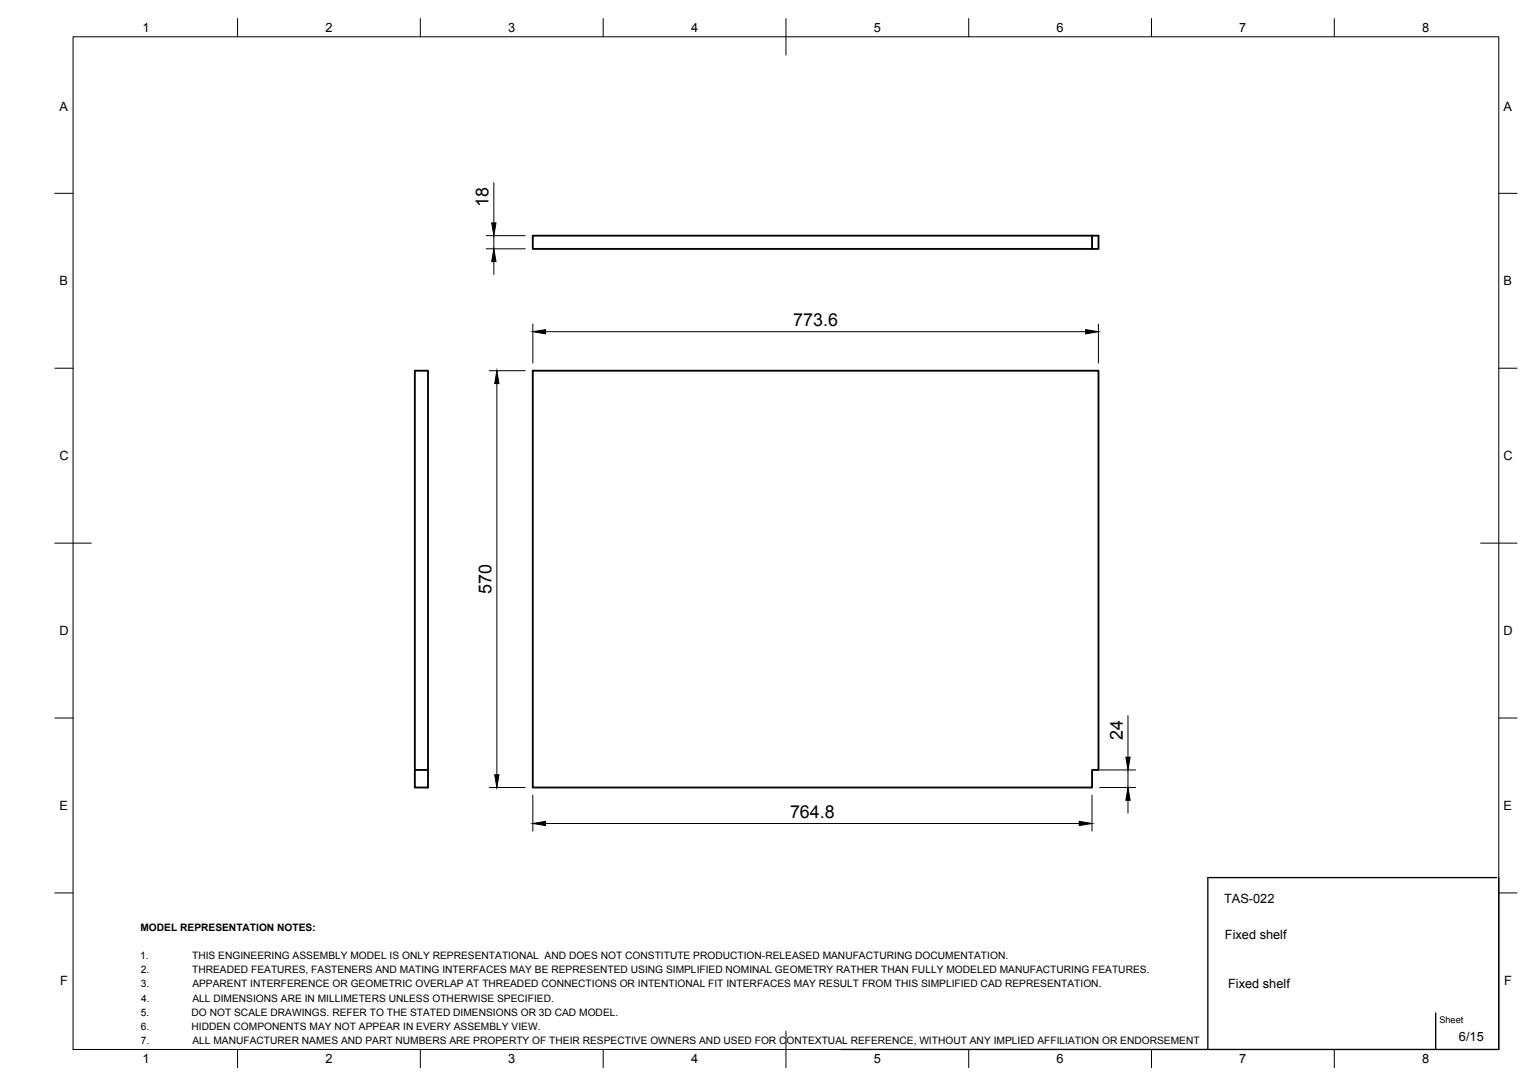
ISO-10303-21;
HEADER;
/* Generated by software containing ST-Developer
 * from STEP Tools, Inc. (www.steptools.com) 
 */

FILE_DESCRIPTION(
/* description */ (''),
/* implementation_level */ '2;1');

FILE_NAME(
/* name */ 'Fixed shelf.step',
/* time_stamp */ '2026-11-15T21:02:08-08:00',
/* author */ (''),
/* organization */ (''),
/* preprocessor_version */ 'ST-DEVELOPER v20.2',
/* originating_system */ 'Autodesk Translation Framework v15.17.0.0',
/* authorisation */ '');

FILE_SCHEMA (('AUTOMOTIVE_DESIGN { 1 0 10303 214 3 1 1 }'));
ENDSEC;

DATA;
#10=MECHANICAL_DESIGN_GEOMETRIC_PRESENTATION_REPRESENTATION('',(#610),#31566);
#580=SHAPE_REPRESENTATION_RELATIONSHIP('SRR','None',#31644,#595);
#595=ADVANCED_BREP_SHAPE_REPRESENTATION('',(#625),#31559);
#610=STYLED_ITEM('',(#31721),#625);
#625=MANIFOLD_SOLID_BREP('Body1',#5723);
#755=FACE_OUTER_BOUND('',#1052,.T.);
#756=FACE_OUTER_BOUND('',#1053,.T.);
#757=FACE_OUTER_BOUND('',#1054,.T.);
#758=FACE_OUTER_BOUND('',#1055,.T.);
#759=FACE_OUTER_BOUND('',#1056,.T.);
#760=FACE_OUTER_BOUND('',#1057,.T.);
#761=FACE_OUTER_BOUND('',#1058,.T.);
#762=FACE_OUTER_BOUND('',#1059,.T.);
#1052=EDGE_LOOP('',(#4245,#4246,#4247,#4248));
#1053=EDGE_LOOP('',(#4249,#4250,#4251,#4252));
#1054=EDGE_LOOP('',(#4253,#4254,#4255,#4256));
#1055=EDGE_LOOP('',(#4257,#4258,#4259,#4260));
#1056=EDGE_LOOP('',(#4261,#4262,#4263,#4264));
#1057=EDGE_LOOP('',(#4265,#4266,#4267,#4268));
#1058=EDGE_LOOP('',(#4269,#4270,#4271,#4272,#4273,#4274));
#1059=EDGE_LOOP('',(#4275,#4276,#4277,#4278,#4279,#4280));
#1463=LINE('',#8212,#1970);
#1464=LINE('',#8214,#1971);
#1465=LINE('',#8216,#1972);
#1466=LINE('',#8217,#1973);
#1467=LINE('',#8220,#1974);
#1468=LINE('',#8222,#1975);
#1469=LINE('',#8223,#1976);
#1470=LINE('',#8226,#1977);
#1471=LINE('',#8228,#1978);
#1472=LINE('',#8229,#1979);
#1473=LINE('',#8232,#1980);
#1474=LINE('',#8234,#1981);
#1475=LINE('',#8235,#1982);
#1476=LINE('',#8238,#1983);
#1477=LINE('',#8240,#1984);
#1478=LINE('',#8241,#1985);
#1479=LINE('',#8243,#1986);
#1480=LINE('',#8244,#1987);
#1970=VECTOR('',#6911,1.);
#1971=VECTOR('',#6912,1.);
#1972=VECTOR('',#6913,1.);
#1973=VECTOR('',#6914,1.);
#1974=VECTOR('',#6917,1.);
#1975=VECTOR('',#6918,1.);
#1976=VECTOR('',#6919,1.);
#1977=VECTOR('',#6922,1.);
#1978=VECTOR('',#6923,1.);
#1979=VECTOR('',#6924,1.);
#1980=VECTOR('',#6927,1.);
#1981=VECTOR('',#6928,1.);
#1982=VECTOR('',#6929,1.);
#1983=VECTOR('',#6932,1.);
#1984=VECTOR('',#6933,1.);
#1985=VECTOR('',#6934,1.);
#1986=VECTOR('',#6937,1.);
#1987=VECTOR('',#6938,1.);
#2426=VERTEX_POINT('',#8210);
#2427=VERTEX_POINT('',#8211);
#2428=VERTEX_POINT('',#8213);
#2429=VERTEX_POINT('',#8215);
#2430=VERTEX_POINT('',#8219);
#2431=VERTEX_POINT('',#8221);
#2432=VERTEX_POINT('',#8225);
#2433=VERTEX_POINT('',#8227);
#2434=VERTEX_POINT('',#8231);
#2435=VERTEX_POINT('',#8233);
#2436=VERTEX_POINT('',#8237);
#2437=VERTEX_POINT('',#8239);
#3118=EDGE_CURVE('',#2426,#2427,#1463,.T.);
#3119=EDGE_CURVE('',#2426,#2428,#1464,.T.);
#3120=EDGE_CURVE('',#2429,#2428,#1465,.T.);
#3121=EDGE_CURVE('',#2427,#2429,#1466,.T.);
#3122=EDGE_CURVE('',#2430,#2426,#1467,.T.);
#3123=EDGE_CURVE('',#2431,#2430,#1468,.T.);
#3124=EDGE_CURVE('',#2428,#2431,#1469,.T.);
#3125=EDGE_CURVE('',#2432,#2429,#1470,.T.);
#3126=EDGE_CURVE('',#2433,#2432,#1471,.T.);
#3127=EDGE_CURVE('',#2433,#2427,#1472,.T.);
#3128=EDGE_CURVE('',#2430,#2434,#1473,.T.);
#3129=EDGE_CURVE('',#2434,#2435,#1474,.T.);
#3130=EDGE_CURVE('',#2431,#2435,#1475,.T.);
#3131=EDGE_CURVE('',#2436,#2433,#1476,.T.);
#3132=EDGE_CURVE('',#2437,#2432,#1477,.T.);
#3133=EDGE_CURVE('',#2436,#2437,#1478,.T.);
#3134=EDGE_CURVE('',#2434,#2436,#1479,.T.);
#3135=EDGE_CURVE('',#2435,#2437,#1480,.T.);
#4245=ORIENTED_EDGE('',*,*,#3118,.F.);
#4246=ORIENTED_EDGE('',*,*,#3119,.T.);
#4247=ORIENTED_EDGE('',*,*,#3120,.F.);
#4248=ORIENTED_EDGE('',*,*,#3121,.F.);
#4249=ORIENTED_EDGE('',*,*,#3122,.F.);
#4250=ORIENTED_EDGE('',*,*,#3123,.F.);
#4251=ORIENTED_EDGE('',*,*,#3124,.F.);
#4252=ORIENTED_EDGE('',*,*,#3119,.F.);
#4253=ORIENTED_EDGE('',*,*,#3121,.T.);
#4254=ORIENTED_EDGE('',*,*,#3125,.F.);
#4255=ORIENTED_EDGE('',*,*,#3126,.F.);
#4256=ORIENTED_EDGE('',*,*,#3127,.T.);
#4257=ORIENTED_EDGE('',*,*,#3123,.T.);
#4258=ORIENTED_EDGE('',*,*,#3128,.T.);
#4259=ORIENTED_EDGE('',*,*,#3129,.T.);
#4260=ORIENTED_EDGE('',*,*,#3130,.F.);
#4261=ORIENTED_EDGE('',*,*,#3131,.T.);
#4262=ORIENTED_EDGE('',*,*,#3126,.T.);
#4263=ORIENTED_EDGE('',*,*,#3132,.F.);
#4264=ORIENTED_EDGE('',*,*,#3133,.F.);
#4265=ORIENTED_EDGE('',*,*,#3134,.T.);
#4266=ORIENTED_EDGE('',*,*,#3133,.T.);
#4267=ORIENTED_EDGE('',*,*,#3135,.F.);
#4268=ORIENTED_EDGE('',*,*,#3129,.F.);
#4269=ORIENTED_EDGE('',*,*,#3124,.T.);
#4270=ORIENTED_EDGE('',*,*,#3130,.T.);
#4271=ORIENTED_EDGE('',*,*,#3135,.T.);
#4272=ORIENTED_EDGE('',*,*,#3132,.T.);
#4273=ORIENTED_EDGE('',*,*,#3125,.T.);
#4274=ORIENTED_EDGE('',*,*,#3120,.T.);
#4275=ORIENTED_EDGE('',*,*,#3118,.T.);
#4276=ORIENTED_EDGE('',*,*,#3127,.F.);
#4277=ORIENTED_EDGE('',*,*,#3131,.F.);
#4278=ORIENTED_EDGE('',*,*,#3134,.F.);
#4279=ORIENTED_EDGE('',*,*,#3128,.F.);
#4280=ORIENTED_EDGE('',*,*,#3122,.T.);
#5360=PLANE('',#6081);
#5361=PLANE('',#6082);
#5362=PLANE('',#6083);
#5363=PLANE('',#6084);
#5364=PLANE('',#6085);
#5365=PLANE('',#6086);
#5366=PLANE('',#6087);
#5367=PLANE('',#6088);
#5569=ADVANCED_FACE('',(#755),#5360,.F.);
#5570=ADVANCED_FACE('',(#756),#5361,.F.);
#5571=ADVANCED_FACE('',(#757),#5362,.T.);
#5572=ADVANCED_FACE('',(#758),#5363,.T.);
#5573=ADVANCED_FACE('',(#759),#5364,.T.);
#5574=ADVANCED_FACE('',(#760),#5365,.T.);
#5575=ADVANCED_FACE('',(#761),#5366,.T.);
#5576=ADVANCED_FACE('',(#762),#5367,.F.);
#5723=CLOSED_SHELL('',(#5569,#5570,#5571,#5572,#5573,#5574,#5575,#5576));
#6080=AXIS2_PLACEMENT_3D('',#8208,#6907,#6908);
#6081=AXIS2_PLACEMENT_3D('',#8209,#6909,#6910);
#6082=AXIS2_PLACEMENT_3D('',#8218,#6915,#6916);
#6083=AXIS2_PLACEMENT_3D('',#8224,#6920,#6921);
#6084=AXIS2_PLACEMENT_3D('',#8230,#6925,#6926);
#6085=AXIS2_PLACEMENT_3D('',#8236,#6930,#6931);
#6086=AXIS2_PLACEMENT_3D('',#8242,#6935,#6936);
#6087=AXIS2_PLACEMENT_3D('',#8245,#6939,#6940);
#6088=AXIS2_PLACEMENT_3D('',#8246,#6941,#6942);
#6907=DIRECTION('axis',(0.,0.,1.));
#6908=DIRECTION('refdir',(1.,0.,0.));
#6909=DIRECTION('center_axis',(0.,1.,0.));
#6910=DIRECTION('ref_axis',(-1.,0.,0.));
#6911=DIRECTION('',(-1.,0.,0.));
#6912=DIRECTION('',(0.,0.,1.));
#6913=DIRECTION('',(1.,0.,0.));
#6914=DIRECTION('',(0.,0.,1.));
#6915=DIRECTION('center_axis',(1.,0.,0.));
#6916=DIRECTION('ref_axis',(0.,1.,0.));
#6917=DIRECTION('',(0.,1.,0.));
#6918=DIRECTION('',(0.,0.,-1.));
#6919=DIRECTION('',(0.,-1.,0.));
#6920=DIRECTION('center_axis',(-1.,0.,0.));
#6921=DIRECTION('ref_axis',(0.,-1.,0.));
#6922=DIRECTION('',(0.,-1.,0.));
#6923=DIRECTION('',(0.,0.,1.));
#6924=DIRECTION('',(0.,-1.,0.));
#6925=DIRECTION('center_axis',(0.,-1.,0.));
#6926=DIRECTION('ref_axis',(1.,0.,0.));
#6927=DIRECTION('',(1.,0.,0.));
#6928=DIRECTION('',(0.,0.,1.));
#6929=DIRECTION('',(1.,0.,0.));
#6930=DIRECTION('center_axis',(0.,1.,0.));
#6931=DIRECTION('ref_axis',(-1.,0.,0.));
#6932=DIRECTION('',(-1.,0.,0.));
#6933=DIRECTION('',(-1.,0.,0.));
#6934=DIRECTION('',(0.,0.,1.));
#6935=DIRECTION('center_axis',(1.,0.,0.));
#6936=DIRECTION('ref_axis',(0.,1.,0.));
#6937=DIRECTION('',(0.,1.,0.));
#6938=DIRECTION('',(0.,1.,0.));
#6939=DIRECTION('center_axis',(0.,0.,1.));
#6940=DIRECTION('ref_axis',(1.,0.,0.));
#6941=DIRECTION('center_axis',(0.,0.,1.));
#6942=DIRECTION('ref_axis',(1.,0.,0.));
#8208=CARTESIAN_POINT('',(0.,0.,0.));
#8209=CARTESIAN_POINT('Origin',(0.88,3.,0.));
#8210=CARTESIAN_POINT('',(0.88,3.,0.));
#8211=CARTESIAN_POINT('',(0.,3.,0.));
#8212=CARTESIAN_POINT('',(19.78,3.,0.));
#8213=CARTESIAN_POINT('',(0.88,3.,1.8));
#8214=CARTESIAN_POINT('',(0.88,3.,0.));
#8215=CARTESIAN_POINT('',(0.,3.,1.8));
#8216=CARTESIAN_POINT('',(19.78,3.,1.8));
#8217=CARTESIAN_POINT('',(0.,3.,0.));
#8218=CARTESIAN_POINT('Origin',(0.88,0.6,0.));
#8219=CARTESIAN_POINT('',(0.88,0.6,0.));
#8220=CARTESIAN_POINT('',(0.880000000000003,14.85,0.));
#8221=CARTESIAN_POINT('',(0.88,0.6,1.8));
#8222=CARTESIAN_POINT('',(0.88,0.6,0.));
#8223=CARTESIAN_POINT('',(0.880000000000003,14.85,1.8));
#8224=CARTESIAN_POINT('Origin',(0.,57.6,0.));
#8225=CARTESIAN_POINT('',(0.,57.6,1.8));
#8226=CARTESIAN_POINT('',(0.,57.6,1.8));
#8227=CARTESIAN_POINT('',(0.,57.6,0.));
#8228=CARTESIAN_POINT('',(0.,57.6,0.));
#8229=CARTESIAN_POINT('',(0.,57.6,0.));
#8230=CARTESIAN_POINT('Origin',(0.,0.6,0.));
#8231=CARTESIAN_POINT('',(77.36,0.6,0.));
#8232=CARTESIAN_POINT('',(0.,0.6,0.));
#8233=CARTESIAN_POINT('',(77.36,0.600000000000001,1.8));
#8234=CARTESIAN_POINT('',(77.36,0.6,0.));
#8235=CARTESIAN_POINT('',(0.,0.6,1.8));
#8236=CARTESIAN_POINT('Origin',(77.36,57.6,0.));
#8237=CARTESIAN_POINT('',(77.36,57.6,0.));
#8238=CARTESIAN_POINT('',(77.36,57.6,0.));
#8239=CARTESIAN_POINT('',(77.36,57.6,1.8));
#8240=CARTESIAN_POINT('',(77.36,57.6,1.8));
#8241=CARTESIAN_POINT('',(77.36,57.6,0.));
#8242=CARTESIAN_POINT('Origin',(77.36,0.6,0.));
#8243=CARTESIAN_POINT('',(77.36,0.6,0.));
#8244=CARTESIAN_POINT('',(77.36,0.6,1.8));
#8245=CARTESIAN_POINT('Origin',(38.68,29.1,1.8));
#8246=CARTESIAN_POINT('Origin',(38.68,29.1,0.));
#31542=UNCERTAINTY_MEASURE_WITH_UNIT(LENGTH_MEASURE(0.001),#31567,
'DISTANCE_ACCURACY_VALUE',
'Maximum model space distance between geometric entities at asserted c
onnectivities');
#31549=UNCERTAINTY_MEASURE_WITH_UNIT(LENGTH_MEASURE(0.001),#31567,
'DISTANCE_ACCURACY_VALUE',
'Maximum model space distance between geometric entities at asserted c
onnectivities');
#31559=(
GEOMETRIC_REPRESENTATION_CONTEXT(3)
GLOBAL_UNCERTAINTY_ASSIGNED_CONTEXT((#31542))
GLOBAL_UNIT_ASSIGNED_CONTEXT((#31567,#31569,#31570))
REPRESENTATION_CONTEXT('','3D')
);
#31566=(
GEOMETRIC_REPRESENTATION_CONTEXT(3)
GLOBAL_UNCERTAINTY_ASSIGNED_CONTEXT((#31549))
GLOBAL_UNIT_ASSIGNED_CONTEXT((#31567,#31569,#31570))
REPRESENTATION_CONTEXT('','3D')
);
#31567=(
LENGTH_UNIT()
NAMED_UNIT(*)
SI_UNIT(.CENTI.,.METRE.)
);
#31569=(
NAMED_UNIT(*)
PLANE_ANGLE_UNIT()
SI_UNIT($,.RADIAN.)
);
#31570=(
NAMED_UNIT(*)
SI_UNIT($,.STERADIAN.)
SOLID_ANGLE_UNIT()
);
#31580=SHAPE_DEFINITION_REPRESENTATION(#31596,#31644);
#31596=PRODUCT_DEFINITION_SHAPE('',$,#31661);
#31644=SHAPE_REPRESENTATION('',(#6080),#31559);
#31651=PRODUCT_DEFINITION_CONTEXT('part definition',#31701,'design');
#31661=PRODUCT_DEFINITION('Fixed shelf','Fixed shelf',#31677,#31651);
#31677=PRODUCT_DEFINITION_FORMATION('',$,#31712);
#31701=APPLICATION_CONTEXT(
'Core Data for Automotive Mechanical Design Process');
#31702=PRODUCT_CONTEXT('part definition',#31701,'mechanical');
#31712=PRODUCT('Fixed shelf','Fixed shelf',$,(#31702));
#31721=PRESENTATION_STYLE_ASSIGNMENT((#31728));
#31728=SURFACE_STYLE_USAGE(.BOTH.,#31735);
#31735=SURFACE_SIDE_STYLE('',(#31742));
#31742=SURFACE_STYLE_FILL_AREA(#31749);
#31749=FILL_AREA_STYLE('Opaque(70,153,204)',(#31756));
#31756=FILL_AREA_STYLE_COLOUR('Opaque(70,153,204)',#31763);
#31763=COLOUR_RGB('Opaque(70,153,204)',0.274509803921569,0.6,0.8);
ENDSEC;
END-ISO-10303-21;
